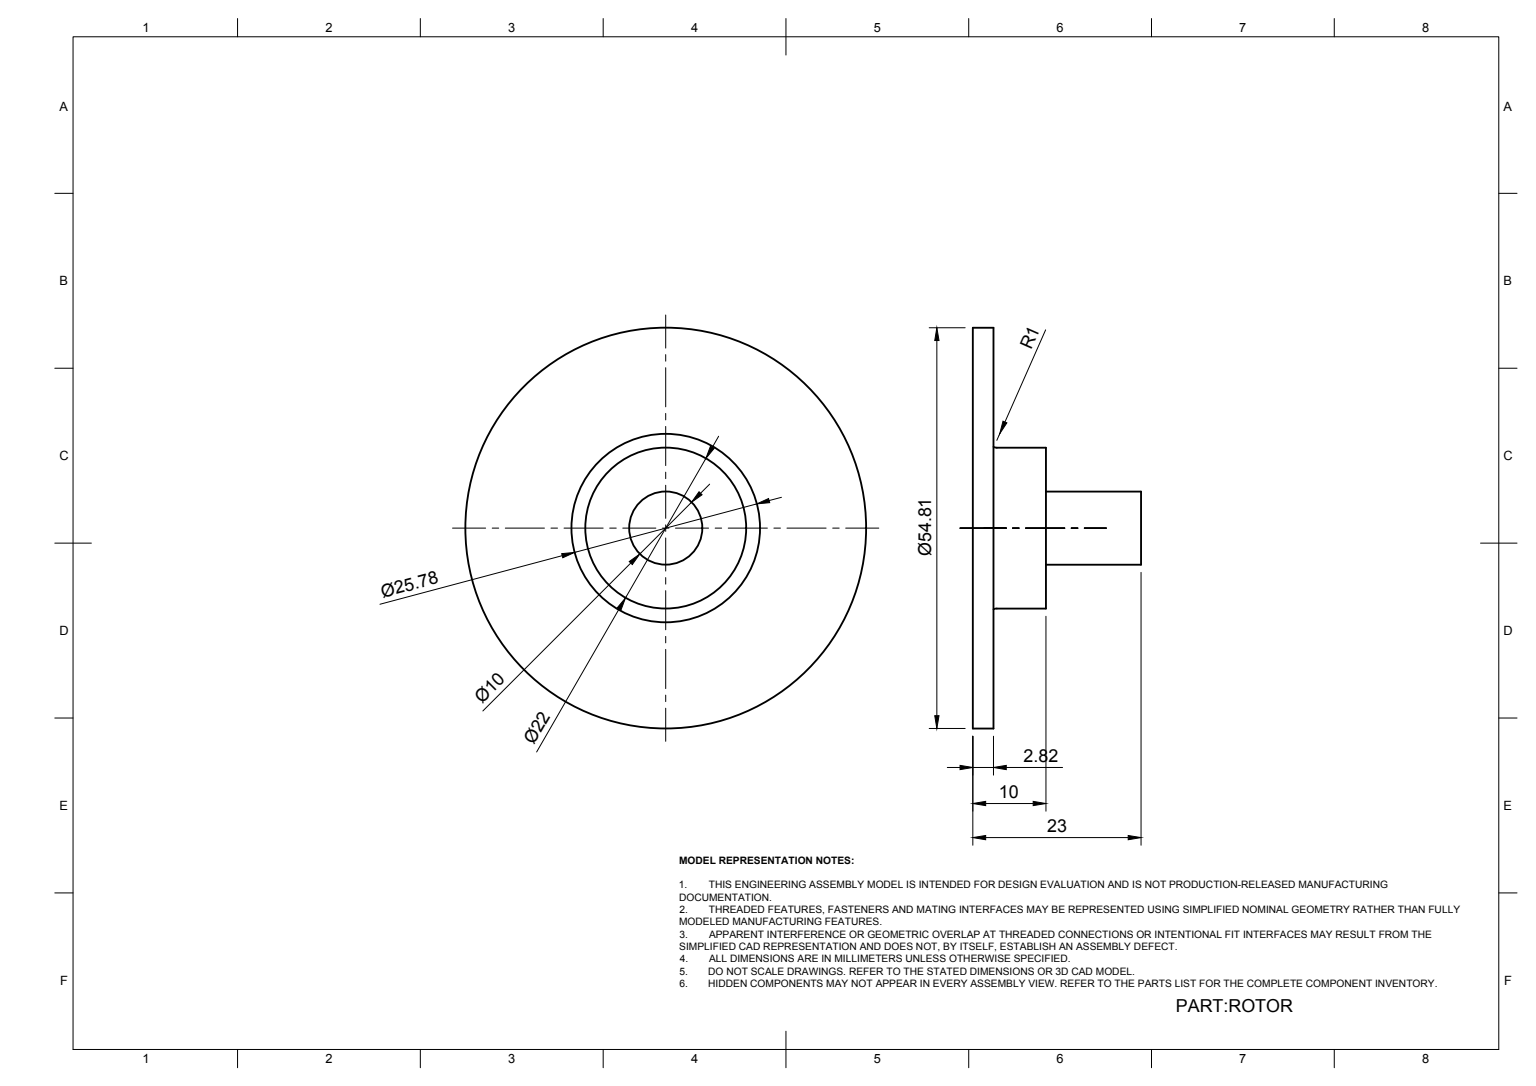
ISO-10303-21;
HEADER;
/* Generated by software containing ST-Developer
 * from STEP Tools, Inc. (www.steptools.com) 
 */

FILE_DESCRIPTION(
/* description */ (''),
/* implementation_level */ '2;1');

FILE_NAME(
/* name */ 'Rotor.step',
/* time_stamp */ '2026-10-04T22:47:03-07:00',
/* author */ (''),
/* organization */ (''),
/* preprocessor_version */ 'ST-DEVELOPER v20.2',
/* originating_system */ 'Autodesk Translation Framework v15.15.0.0',
/* authorisation */ '');

FILE_SCHEMA (('AUTOMOTIVE_DESIGN { 1 0 10303 214 3 1 1 }'));
ENDSEC;

DATA;
#10=MECHANICAL_DESIGN_GEOMETRIC_PRESENTATION_REPRESENTATION('',(#80),#19878);
#45=TOROIDAL_SURFACE('',#5257,12.,1.);
#66=SHAPE_REPRESENTATION_RELATIONSHIP('SRR','None',#19910,#73);
#73=ADVANCED_BREP_SHAPE_REPRESENTATION('',(#87),#19874);
#80=STYLED_ITEM('',(#19953),#87);
#87=MANIFOLD_SOLID_BREP('Body1',#4828);
#95=FACE_BOUND('',#808,.T.);
#96=FACE_BOUND('',#814,.T.);
#301=PLANE('',#5255);
#302=PLANE('',#5262);
#303=PLANE('',#5266);
#304=PLANE('',#5267);
#526=FACE_OUTER_BOUND('',#806,.T.);
#527=FACE_OUTER_BOUND('',#807,.T.);
#528=FACE_OUTER_BOUND('',#809,.T.);
#529=FACE_OUTER_BOUND('',#810,.T.);
#530=FACE_OUTER_BOUND('',#811,.T.);
#531=FACE_OUTER_BOUND('',#812,.T.);
#532=FACE_OUTER_BOUND('',#813,.T.);
#533=FACE_OUTER_BOUND('',#815,.T.);
#806=EDGE_LOOP('',(#4133,#4134,#4135,#4136));
#807=EDGE_LOOP('',(#4137));
#808=EDGE_LOOP('',(#4138));
#809=EDGE_LOOP('',(#4139,#4140,#4141,#4142));
#810=EDGE_LOOP('',(#4143,#4144,#4145,#4146));
#811=EDGE_LOOP('',(#4147));
#812=EDGE_LOOP('',(#4148,#4149,#4150,#4151));
#813=EDGE_LOOP('',(#4152));
#814=EDGE_LOOP('',(#4153));
#815=EDGE_LOOP('',(#4154));
#1194=LINE('',#19541,#1550);
#1195=LINE('',#19553,#1551);
#1196=LINE('',#19560,#1552);
#1550=VECTOR('',#6412,5.);
#1551=VECTOR('',#6429,11.);
#1552=VECTOR('',#6438,27.4027293621977);
#1785=CIRCLE('',#5253,5.);
#1786=CIRCLE('',#5254,5.);
#1787=CIRCLE('',#5256,11.);
#1788=CIRCLE('',#5258,11.);
#1789=CIRCLE('',#5259,1.);
#1790=CIRCLE('',#5260,12.8892103004758);
#1791=CIRCLE('',#5263,27.4027293621977);
#1792=CIRCLE('',#5265,27.4027293621977);
#2235=VERTEX_POINT('',#19538);
#2236=VERTEX_POINT('',#19540);
#2237=VERTEX_POINT('',#19544);
#2238=VERTEX_POINT('',#19547);
#2239=VERTEX_POINT('',#19549);
#2240=VERTEX_POINT('',#19555);
#2241=VERTEX_POINT('',#19558);
#2878=EDGE_CURVE('',#2235,#2235,#1785,.T.);
#2879=EDGE_CURVE('',#2235,#2236,#1194,.T.);
#2880=EDGE_CURVE('',#2236,#2236,#1786,.T.);
#2881=EDGE_CURVE('',#2237,#2237,#1787,.T.);
#2882=EDGE_CURVE('',#2238,#2238,#1788,.T.);
#2883=EDGE_CURVE('',#2238,#2239,#1789,.T.);
#2884=EDGE_CURVE('',#2239,#2239,#1790,.T.);
#2885=EDGE_CURVE('',#2237,#2238,#1195,.T.);
#2886=EDGE_CURVE('',#2240,#2240,#1791,.T.);
#2887=EDGE_CURVE('',#2241,#2241,#1792,.T.);
#2888=EDGE_CURVE('',#2241,#2240,#1196,.T.);
#4133=ORIENTED_EDGE('',*,*,#2878,.T.);
#4134=ORIENTED_EDGE('',*,*,#2879,.T.);
#4135=ORIENTED_EDGE('',*,*,#2880,.F.);
#4136=ORIENTED_EDGE('',*,*,#2879,.F.);
#4137=ORIENTED_EDGE('',*,*,#2881,.T.);
#4138=ORIENTED_EDGE('',*,*,#2878,.F.);
#4139=ORIENTED_EDGE('',*,*,#2882,.F.);
#4140=ORIENTED_EDGE('',*,*,#2883,.T.);
#4141=ORIENTED_EDGE('',*,*,#2884,.T.);
#4142=ORIENTED_EDGE('',*,*,#2883,.F.);
#4143=ORIENTED_EDGE('',*,*,#2881,.F.);
#4144=ORIENTED_EDGE('',*,*,#2885,.T.);
#4145=ORIENTED_EDGE('',*,*,#2882,.T.);
#4146=ORIENTED_EDGE('',*,*,#2885,.F.);
#4147=ORIENTED_EDGE('',*,*,#2886,.F.);
#4148=ORIENTED_EDGE('',*,*,#2887,.F.);
#4149=ORIENTED_EDGE('',*,*,#2888,.T.);
#4150=ORIENTED_EDGE('',*,*,#2886,.T.);
#4151=ORIENTED_EDGE('',*,*,#2888,.F.);
#4152=ORIENTED_EDGE('',*,*,#2887,.T.);
#4153=ORIENTED_EDGE('',*,*,#2884,.F.);
#4154=ORIENTED_EDGE('',*,*,#2880,.T.);
#4516=CYLINDRICAL_SURFACE('',#5252,5.);
#4517=CYLINDRICAL_SURFACE('',#5261,11.);
#4518=CYLINDRICAL_SURFACE('',#5264,27.4027293621977);
#4750=ADVANCED_FACE('',(#526),#4516,.T.);
#4751=ADVANCED_FACE('',(#527,#95),#301,.T.);
#4752=ADVANCED_FACE('',(#528),#45,.F.);
#4753=ADVANCED_FACE('',(#529),#4517,.T.);
#4754=ADVANCED_FACE('',(#530),#302,.T.);
#4755=ADVANCED_FACE('',(#531),#4518,.T.);
#4756=ADVANCED_FACE('',(#532,#96),#303,.T.);
#4757=ADVANCED_FACE('',(#533),#304,.T.);
#4828=CLOSED_SHELL('',(#4750,#4751,#4752,#4753,#4754,#4755,#4756,#4757));
#5251=AXIS2_PLACEMENT_3D('',#19536,#6406,#6407);
#5252=AXIS2_PLACEMENT_3D('',#19537,#6408,#6409);
#5253=AXIS2_PLACEMENT_3D('',#19539,#6410,#6411);
#5254=AXIS2_PLACEMENT_3D('',#19542,#6413,#6414);
#5255=AXIS2_PLACEMENT_3D('',#19543,#6415,#6416);
#5256=AXIS2_PLACEMENT_3D('',#19545,#6417,#6418);
#5257=AXIS2_PLACEMENT_3D('',#19546,#6419,#6420);
#5258=AXIS2_PLACEMENT_3D('',#19548,#6421,#6422);
#5259=AXIS2_PLACEMENT_3D('',#19550,#6423,#6424);
#5260=AXIS2_PLACEMENT_3D('',#19551,#6425,#6426);
#5261=AXIS2_PLACEMENT_3D('',#19552,#6427,#6428);
#5262=AXIS2_PLACEMENT_3D('',#19554,#6430,#6431);
#5263=AXIS2_PLACEMENT_3D('',#19556,#6432,#6433);
#5264=AXIS2_PLACEMENT_3D('',#19557,#6434,#6435);
#5265=AXIS2_PLACEMENT_3D('',#19559,#6436,#6437);
#5266=AXIS2_PLACEMENT_3D('',#19561,#6439,#6440);
#5267=AXIS2_PLACEMENT_3D('',#19562,#6441,#6442);
#6406=DIRECTION('axis',(0.,0.,1.));
#6407=DIRECTION('refdir',(1.,0.,0.));
#6408=DIRECTION('center_axis',(0.,0.,-1.));
#6409=DIRECTION('ref_axis',(-1.,0.,0.));
#6410=DIRECTION('center_axis',(0.,0.,1.));
#6411=DIRECTION('ref_axis',(-1.,0.,0.));
#6412=DIRECTION('',(0.,0.,1.));
#6413=DIRECTION('center_axis',(0.,0.,1.));
#6414=DIRECTION('ref_axis',(-1.,0.,0.));
#6415=DIRECTION('center_axis',(0.,0.,1.));
#6416=DIRECTION('ref_axis',(1.,0.,0.));
#6417=DIRECTION('center_axis',(0.,0.,1.));
#6418=DIRECTION('ref_axis',(1.,0.,0.));
#6419=DIRECTION('center_axis',(0.,0.,1.));
#6420=DIRECTION('ref_axis',(1.,0.,0.));
#6421=DIRECTION('center_axis',(0.,0.,1.));
#6422=DIRECTION('ref_axis',(1.,0.,0.));
#6423=DIRECTION('center_axis',(-1.22464679914735E-16,1.,0.));
#6424=DIRECTION('ref_axis',(-1.,-1.22464679914735E-16,0.));
#6425=DIRECTION('center_axis',(0.,0.,1.));
#6426=DIRECTION('ref_axis',(1.,0.,0.));
#6427=DIRECTION('center_axis',(0.,0.,1.));
#6428=DIRECTION('ref_axis',(1.,0.,0.));
#6429=DIRECTION('',(0.,0.,-1.));
#6430=DIRECTION('center_axis',(0.,0.,-1.));
#6431=DIRECTION('ref_axis',(-1.,0.,0.));
#6432=DIRECTION('center_axis',(0.,0.,1.));
#6433=DIRECTION('ref_axis',(1.,0.,0.));
#6434=DIRECTION('center_axis',(0.,0.,1.));
#6435=DIRECTION('ref_axis',(1.,0.,0.));
#6436=DIRECTION('center_axis',(0.,0.,1.));
#6437=DIRECTION('ref_axis',(1.,0.,0.));
#6438=DIRECTION('',(0.,0.,-1.));
#6439=DIRECTION('center_axis',(0.,0.,1.));
#6440=DIRECTION('ref_axis',(1.,0.,0.));
#6441=DIRECTION('center_axis',(0.,0.,1.));
#6442=DIRECTION('ref_axis',(-1.,0.,0.));
#19536=CARTESIAN_POINT('',(0.,0.,0.));
#19537=CARTESIAN_POINT('Origin',(0.,0.,13.));
#19538=CARTESIAN_POINT('',(5.,6.12323399573677E-16,0.));
#19539=CARTESIAN_POINT('Origin',(0.,0.,0.));
#19540=CARTESIAN_POINT('',(5.,6.12323399573677E-16,13.));
#19541=CARTESIAN_POINT('',(5.,-6.12323399573677E-16,13.));
#19542=CARTESIAN_POINT('Origin',(0.,0.,13.));
#19543=CARTESIAN_POINT('Origin',(0.,0.,0.));
#19544=CARTESIAN_POINT('',(-11.,-1.34711147906209E-15,0.));
#19545=CARTESIAN_POINT('Origin',(0.,0.,0.));
#19546=CARTESIAN_POINT('Origin',(0.,0.,-6.72261291411212));
#19547=CARTESIAN_POINT('',(-11.,-1.34711147906209E-15,-6.72261291411212));
#19548=CARTESIAN_POINT('Origin',(0.,0.,-6.72261291411212));
#19549=CARTESIAN_POINT('',(-12.8892103004758,-1.57847301380148E-15,-7.18011159337554));
#19550=CARTESIAN_POINT('Origin',(-12.,-1.46957615897682E-15,-6.72261291411212));
#19551=CARTESIAN_POINT('Origin',(0.,0.,-7.18011159337554));
#19552=CARTESIAN_POINT('Origin',(0.,0.,-3.36130645705606));
#19553=CARTESIAN_POINT('',(-11.,-1.34711147906209E-15,-3.36130645705606));
#19554=CARTESIAN_POINT('Origin',(27.4027293621977,0.,-10.));
#19555=CARTESIAN_POINT('',(-27.4027293621977,-3.35586648013166E-15,-10.));
#19556=CARTESIAN_POINT('Origin',(0.,0.,-10.));
#19557=CARTESIAN_POINT('Origin',(0.,0.,-8.59005579668777));
#19558=CARTESIAN_POINT('',(-27.4027293621977,-3.35586648013166E-15,-7.18011159337554));
#19559=CARTESIAN_POINT('Origin',(0.,0.,-7.18011159337554));
#19560=CARTESIAN_POINT('',(-27.4027293621977,-3.35586648013166E-15,-8.59005579668777));
#19561=CARTESIAN_POINT('Origin',(12.8892103004758,0.,-7.18011159337554));
#19562=CARTESIAN_POINT('Origin',(0.,2.22044604925031E-15,13.));
#19865=UNCERTAINTY_MEASURE_WITH_UNIT(LENGTH_MEASURE(0.01),#19879,
'DISTANCE_ACCURACY_VALUE',
'Maximum model space distance between geometric entities at asserted c
onnectivities');
#19869=UNCERTAINTY_MEASURE_WITH_UNIT(LENGTH_MEASURE(0.01),#19879,
'DISTANCE_ACCURACY_VALUE',
'Maximum model space distance between geometric entities at asserted c
onnectivities');
#19874=(
GEOMETRIC_REPRESENTATION_CONTEXT(3)
GLOBAL_UNCERTAINTY_ASSIGNED_CONTEXT((#19865))
GLOBAL_UNIT_ASSIGNED_CONTEXT((#19879,#19881,#19882))
REPRESENTATION_CONTEXT('','3D')
);
#19878=(
GEOMETRIC_REPRESENTATION_CONTEXT(3)
GLOBAL_UNCERTAINTY_ASSIGNED_CONTEXT((#19869))
GLOBAL_UNIT_ASSIGNED_CONTEXT((#19879,#19881,#19882))
REPRESENTATION_CONTEXT('','3D')
);
#19879=(
LENGTH_UNIT()
NAMED_UNIT(*)
SI_UNIT(.MILLI.,.METRE.)
);
#19881=(
NAMED_UNIT(*)
PLANE_ANGLE_UNIT()
SI_UNIT($,.RADIAN.)
);
#19882=(
NAMED_UNIT(*)
SI_UNIT($,.STERADIAN.)
SOLID_ANGLE_UNIT()
);
#19887=SHAPE_DEFINITION_REPRESENTATION(#19895,#19910);
#19895=PRODUCT_DEFINITION_SHAPE('',$,#19919);
#19910=SHAPE_REPRESENTATION('',(#5251),#19874);
#19914=PRODUCT_DEFINITION_CONTEXT('part definition',#19940,'design');
#19919=PRODUCT_DEFINITION('Rotor','Rotor',#19927,#19914);
#19927=PRODUCT_DEFINITION_FORMATION('',$,#19946);
#19940=APPLICATION_CONTEXT(
'Core Data for Automotive Mechanical Design Process');
#19941=PRODUCT_CONTEXT('part definition',#19940,'mechanical');
#19946=PRODUCT('Rotor','Rotor',$,(#19941));
#19953=PRESENTATION_STYLE_ASSIGNMENT((#19959));
#19959=SURFACE_STYLE_USAGE(.BOTH.,#19965);
#19965=SURFACE_SIDE_STYLE('',(#19971));
#19971=SURFACE_STYLE_FILL_AREA(#19977);
#19977=FILL_AREA_STYLE('Opaque(255,85,127)',(#19983));
#19983=FILL_AREA_STYLE_COLOUR('Opaque(255,85,127)',#19989);
#19989=COLOUR_RGB('Opaque(255,85,127)', 0.40784314, 0.44705882, 0.49803922);
ENDSEC;
END-ISO-10303-21;
